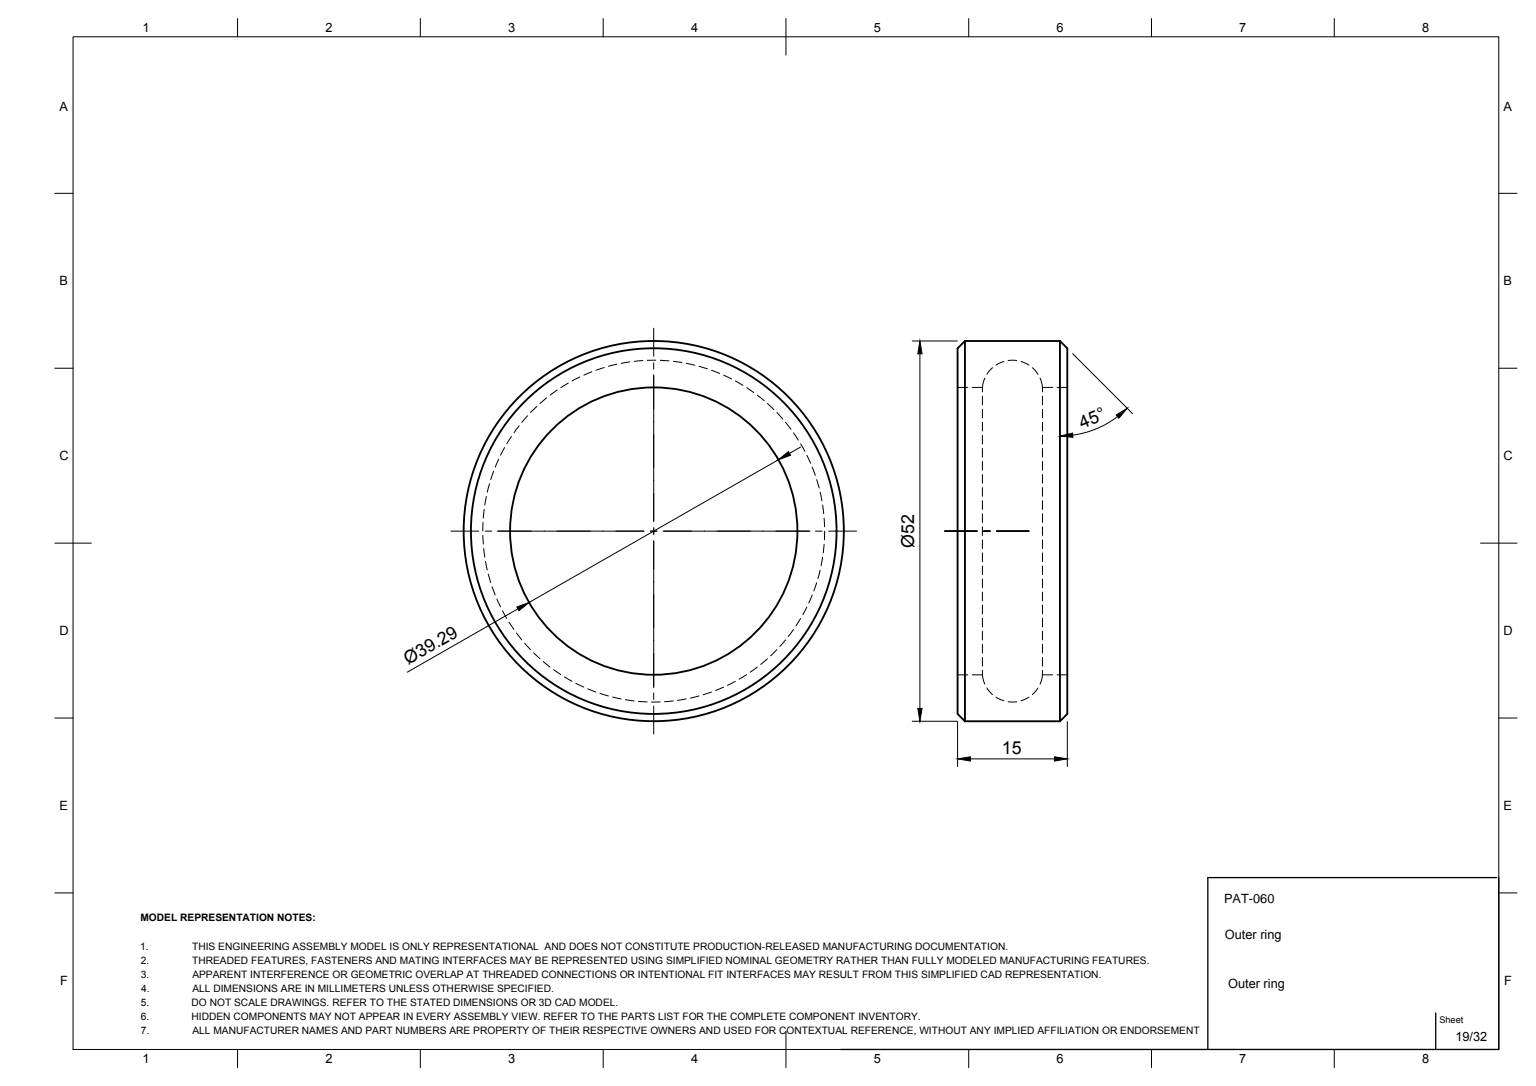
ISO-10303-21;
HEADER;
/* Generated by software containing ST-Developer
 * from STEP Tools, Inc. (www.steptools.com) 
 */

FILE_DESCRIPTION(
/* description */ ('Indexing fixture plate with plunger'),
/* implementation_level */ '2;1');

FILE_NAME(
/* name */ 'Outer ring.step',
/* time_stamp */ '2026-10-28T03:23:41-07:00',
/* author */ (''),
/* organization */ (''),
/* preprocessor_version */ 'ST-DEVELOPER v20.2',
/* originating_system */ 'Autodesk Translation Framework v15.17.0.0',
/* authorisation */ '');

FILE_SCHEMA (('AUTOMOTIVE_DESIGN { 1 0 10303 214 3 1 1 }'));
ENDSEC;

DATA;
#10=MECHANICAL_DESIGN_GEOMETRIC_PRESENTATION_REPRESENTATION('',(#331),#10020);
#214=TOROIDAL_SURFACE('',#5106,1.925,0.412776);
#220=CONICAL_SURFACE('',#5117,2.55,0.785398163397449);
#221=CONICAL_SURFACE('',#5121,2.55,0.785398163397449);
#277=SHAPE_REPRESENTATION_RELATIONSHIP('SRR','None',#10152,#304);
#304=ADVANCED_BREP_SHAPE_REPRESENTATION('',(#366),#10005);
#331=STYLED_ITEM('',(#10368),#366);
#366=MANIFOLD_SOLID_BREP('Body1',#4586);
#433=FACE_BOUND('',#1099,.T.);
#434=FACE_BOUND('',#1104,.T.);
#585=PLANE('',#5114);
#586=PLANE('',#5123);
#764=FACE_OUTER_BOUND('',#1096,.T.);
#765=FACE_OUTER_BOUND('',#1097,.T.);
#766=FACE_OUTER_BOUND('',#1098,.T.);
#767=FACE_OUTER_BOUND('',#1100,.T.);
#768=FACE_OUTER_BOUND('',#1101,.T.);
#769=FACE_OUTER_BOUND('',#1102,.T.);
#770=FACE_OUTER_BOUND('',#1103,.T.);
#771=FACE_OUTER_BOUND('',#1105,.T.);
#1096=EDGE_LOOP('',(#3403,#3404,#3405,#3406,#3407,#3408));
#1097=EDGE_LOOP('',(#3409,#3410,#3411,#3412,#3413));
#1098=EDGE_LOOP('',(#3414));
#1099=EDGE_LOOP('',(#3415));
#1100=EDGE_LOOP('',(#3416,#3417,#3418,#3419));
#1101=EDGE_LOOP('',(#3420,#3421,#3422,#3423));
#1102=EDGE_LOOP('',(#3424,#3425,#3426,#3427));
#1103=EDGE_LOOP('',(#3428));
#1104=EDGE_LOOP('',(#3429));
#1105=EDGE_LOOP('',(#3430,#3431,#3432,#3433,#3434));
#1468=LINE('',#8647,#1688);
#1469=LINE('',#8656,#1689);
#1470=LINE('',#8660,#1690);
#1471=LINE('',#8664,#1691);
#1472=LINE('',#8667,#1692);
#1688=VECTOR('',#6063,1.96469);
#1689=VECTOR('',#6074,2.55);
#1690=VECTOR('',#6079,2.6);
#1691=VECTOR('',#6084,2.55);
#1692=VECTOR('',#6089,1.96469);
#1920=CIRCLE('',#5107,1.96469);
#1921=CIRCLE('',#5108,1.96469);
#1922=CIRCLE('',#5109,0.412776);
#1923=CIRCLE('',#5110,1.96469);
#1924=CIRCLE('',#5111,1.96469);
#1925=CIRCLE('',#5113,1.96469);
#1926=CIRCLE('',#5115,2.5);
#1927=CIRCLE('',#5116,1.96469);
#1928=CIRCLE('',#5118,2.6);
#1929=CIRCLE('',#5120,2.6);
#1930=CIRCLE('',#5122,2.5);
#2247=VERTEX_POINT('',#8635);
#2248=VERTEX_POINT('',#8636);
#2249=VERTEX_POINT('',#8639);
#2250=VERTEX_POINT('',#8641);
#2251=VERTEX_POINT('',#8645);
#2252=VERTEX_POINT('',#8649);
#2253=VERTEX_POINT('',#8651);
#2254=VERTEX_POINT('',#8654);
#2255=VERTEX_POINT('',#8658);
#2256=VERTEX_POINT('',#8662);
#2681=EDGE_CURVE('',#2247,#2248,#1920,.T.);
#2682=EDGE_CURVE('',#2248,#2247,#1921,.T.);
#2683=EDGE_CURVE('',#2248,#2249,#1922,.T.);
#2684=EDGE_CURVE('',#2250,#2249,#1923,.T.);
#2685=EDGE_CURVE('',#2249,#2250,#1924,.T.);
#2686=EDGE_CURVE('',#2251,#2251,#1925,.T.);
#2687=EDGE_CURVE('',#2251,#2250,#1468,.T.);
#2688=EDGE_CURVE('',#2252,#2252,#1926,.T.);
#2689=EDGE_CURVE('',#2253,#2253,#1927,.T.);
#2690=EDGE_CURVE('',#2254,#2254,#1928,.T.);
#2691=EDGE_CURVE('',#2254,#2252,#1469,.T.);
#2692=EDGE_CURVE('',#2255,#2255,#1929,.T.);
#2693=EDGE_CURVE('',#2255,#2254,#1470,.T.);
#2694=EDGE_CURVE('',#2256,#2256,#1930,.T.);
#2695=EDGE_CURVE('',#2256,#2255,#1471,.T.);
#2696=EDGE_CURVE('',#2247,#2253,#1472,.T.);
#3403=ORIENTED_EDGE('',*,*,#2681,.F.);
#3404=ORIENTED_EDGE('',*,*,#2682,.F.);
#3405=ORIENTED_EDGE('',*,*,#2683,.T.);
#3406=ORIENTED_EDGE('',*,*,#2684,.F.);
#3407=ORIENTED_EDGE('',*,*,#2685,.F.);
#3408=ORIENTED_EDGE('',*,*,#2683,.F.);
#3409=ORIENTED_EDGE('',*,*,#2686,.T.);
#3410=ORIENTED_EDGE('',*,*,#2687,.T.);
#3411=ORIENTED_EDGE('',*,*,#2684,.T.);
#3412=ORIENTED_EDGE('',*,*,#2685,.T.);
#3413=ORIENTED_EDGE('',*,*,#2687,.F.);
#3414=ORIENTED_EDGE('',*,*,#2688,.F.);
#3415=ORIENTED_EDGE('',*,*,#2689,.T.);
#3416=ORIENTED_EDGE('',*,*,#2690,.F.);
#3417=ORIENTED_EDGE('',*,*,#2691,.T.);
#3418=ORIENTED_EDGE('',*,*,#2688,.T.);
#3419=ORIENTED_EDGE('',*,*,#2691,.F.);
#3420=ORIENTED_EDGE('',*,*,#2692,.F.);
#3421=ORIENTED_EDGE('',*,*,#2693,.T.);
#3422=ORIENTED_EDGE('',*,*,#2690,.T.);
#3423=ORIENTED_EDGE('',*,*,#2693,.F.);
#3424=ORIENTED_EDGE('',*,*,#2694,.F.);
#3425=ORIENTED_EDGE('',*,*,#2695,.T.);
#3426=ORIENTED_EDGE('',*,*,#2692,.T.);
#3427=ORIENTED_EDGE('',*,*,#2695,.F.);
#3428=ORIENTED_EDGE('',*,*,#2694,.T.);
#3429=ORIENTED_EDGE('',*,*,#2686,.F.);
#3430=ORIENTED_EDGE('',*,*,#2681,.T.);
#3431=ORIENTED_EDGE('',*,*,#2682,.T.);
#3432=ORIENTED_EDGE('',*,*,#2696,.T.);
#3433=ORIENTED_EDGE('',*,*,#2689,.F.);
#3434=ORIENTED_EDGE('',*,*,#2696,.F.);
#4206=CYLINDRICAL_SURFACE('',#5112,1.96469);
#4207=CYLINDRICAL_SURFACE('',#5119,2.6);
#4208=CYLINDRICAL_SURFACE('',#5124,1.96469);
#4379=ADVANCED_FACE('',(#764),#214,.F.);
#4380=ADVANCED_FACE('',(#765),#4206,.F.);
#4381=ADVANCED_FACE('',(#766,#433),#585,.T.);
#4382=ADVANCED_FACE('',(#767),#220,.T.);
#4383=ADVANCED_FACE('',(#768),#4207,.T.);
#4384=ADVANCED_FACE('',(#769),#221,.T.);
#4385=ADVANCED_FACE('',(#770,#434),#586,.T.);
#4386=ADVANCED_FACE('',(#771),#4208,.F.);
#4586=CLOSED_SHELL('',(#4379,#4380,#4381,#4382,#4383,#4384,#4385,#4386));
#5105=AXIS2_PLACEMENT_3D('',#8633,#6045,#6046);
#5106=AXIS2_PLACEMENT_3D('',#8634,#6047,#6048);
#5107=AXIS2_PLACEMENT_3D('',#8637,#6049,#6050);
#5108=AXIS2_PLACEMENT_3D('',#8638,#6051,#6052);
#5109=AXIS2_PLACEMENT_3D('',#8640,#6053,#6054);
#5110=AXIS2_PLACEMENT_3D('',#8642,#6055,#6056);
#5111=AXIS2_PLACEMENT_3D('',#8643,#6057,#6058);
#5112=AXIS2_PLACEMENT_3D('',#8644,#6059,#6060);
#5113=AXIS2_PLACEMENT_3D('',#8646,#6061,#6062);
#5114=AXIS2_PLACEMENT_3D('',#8648,#6064,#6065);
#5115=AXIS2_PLACEMENT_3D('',#8650,#6066,#6067);
#5116=AXIS2_PLACEMENT_3D('',#8652,#6068,#6069);
#5117=AXIS2_PLACEMENT_3D('',#8653,#6070,#6071);
#5118=AXIS2_PLACEMENT_3D('',#8655,#6072,#6073);
#5119=AXIS2_PLACEMENT_3D('',#8657,#6075,#6076);
#5120=AXIS2_PLACEMENT_3D('',#8659,#6077,#6078);
#5121=AXIS2_PLACEMENT_3D('',#8661,#6080,#6081);
#5122=AXIS2_PLACEMENT_3D('',#8663,#6082,#6083);
#5123=AXIS2_PLACEMENT_3D('',#8665,#6085,#6086);
#5124=AXIS2_PLACEMENT_3D('',#8666,#6087,#6088);
#6045=DIRECTION('axis',(0.,0.,1.));
#6046=DIRECTION('refdir',(1.,0.,0.));
#6047=DIRECTION('center_axis',(0.,-1.,0.));
#6048=DIRECTION('ref_axis',(0.,0.,-1.));
#6049=DIRECTION('center_axis',(0.,-1.,0.));
#6050=DIRECTION('ref_axis',(1.,0.,0.));
#6051=DIRECTION('center_axis',(0.,-1.,0.));
#6052=DIRECTION('ref_axis',(1.,0.,0.));
#6053=DIRECTION('center_axis',(1.,0.,1.22464679914735E-16));
#6054=DIRECTION('ref_axis',(-1.22464679914735E-16,0.,1.));
#6055=DIRECTION('center_axis',(0.,1.,0.));
#6056=DIRECTION('ref_axis',(1.,0.,0.));
#6057=DIRECTION('center_axis',(0.,1.,0.));
#6058=DIRECTION('ref_axis',(1.,0.,0.));
#6059=DIRECTION('center_axis',(0.,-1.,0.));
#6060=DIRECTION('ref_axis',(1.,0.,0.));
#6061=DIRECTION('center_axis',(0.,-1.,0.));
#6062=DIRECTION('ref_axis',(1.,0.,0.));
#6063=DIRECTION('',(0.,1.,0.));
#6064=DIRECTION('center_axis',(0.,1.,0.));
#6065=DIRECTION('ref_axis',(0.,0.,1.));
#6066=DIRECTION('center_axis',(0.,-1.,0.));
#6067=DIRECTION('ref_axis',(1.,0.,0.));
#6068=DIRECTION('center_axis',(0.,-1.,0.));
#6069=DIRECTION('ref_axis',(1.,0.,0.));
#6070=DIRECTION('center_axis',(0.,-1.,0.));
#6071=DIRECTION('ref_axis',(1.,0.,0.));
#6072=DIRECTION('center_axis',(0.,-1.,0.));
#6073=DIRECTION('ref_axis',(1.,0.,0.));
#6074=DIRECTION('',(0.707106781186548,0.707106781186547,8.65956056235494E-17));
#6075=DIRECTION('center_axis',(0.,-1.,0.));
#6076=DIRECTION('ref_axis',(1.,0.,0.));
#6077=DIRECTION('center_axis',(0.,-1.,0.));
#6078=DIRECTION('ref_axis',(1.,0.,0.));
#6079=DIRECTION('',(0.,1.,0.));
#6080=DIRECTION('center_axis',(0.,1.,0.));
#6081=DIRECTION('ref_axis',(1.,0.,0.));
#6082=DIRECTION('center_axis',(0.,-1.,0.));
#6083=DIRECTION('ref_axis',(1.,0.,0.));
#6084=DIRECTION('',(-0.707106781186548,0.707106781186547,-8.65956056235494E-17));
#6085=DIRECTION('center_axis',(0.,-1.,0.));
#6086=DIRECTION('ref_axis',(0.,0.,-1.));
#6087=DIRECTION('center_axis',(0.,-1.,0.));
#6088=DIRECTION('ref_axis',(1.,0.,0.));
#6089=DIRECTION('',(0.,1.,0.));
#8633=CARTESIAN_POINT('',(0.,0.,0.));
#8634=CARTESIAN_POINT('Origin',(0.,0.,0.));
#8635=CARTESIAN_POINT('',(-1.96469,0.410863395882378,-2.40605131981681E-16));
#8636=CARTESIAN_POINT('',(-2.40605131981681E-16,0.410863395882378,1.96469));
#8637=CARTESIAN_POINT('Origin',(0.,0.410863395882378,0.));
#8638=CARTESIAN_POINT('Origin',(0.,0.410863395882378,0.));
#8639=CARTESIAN_POINT('',(-2.40605131981681E-16,-0.410863395882378,1.96469));
#8640=CARTESIAN_POINT('Origin',(-2.35744508835865E-16,0.,1.925));
#8641=CARTESIAN_POINT('',(-1.96469,-0.410863395882378,2.40605131981681E-16));
#8642=CARTESIAN_POINT('Origin',(0.,-0.410863395882378,0.));
#8643=CARTESIAN_POINT('Origin',(0.,-0.410863395882378,0.));
#8644=CARTESIAN_POINT('Origin',(0.,0.,0.));
#8645=CARTESIAN_POINT('',(-1.96469,-0.75,-2.40605131981681E-16));
#8646=CARTESIAN_POINT('Origin',(0.,-0.75,0.));
#8647=CARTESIAN_POINT('',(-1.96469,0.,-2.40605131981681E-16));
#8648=CARTESIAN_POINT('Origin',(2.5,0.75,0.));
#8649=CARTESIAN_POINT('',(-2.5,0.75,-3.06161699786838E-16));
#8650=CARTESIAN_POINT('Origin',(0.,0.75,0.));
#8651=CARTESIAN_POINT('',(-1.96469,0.75,-2.40605131981681E-16));
#8652=CARTESIAN_POINT('Origin',(0.,0.75,0.));
#8653=CARTESIAN_POINT('Origin',(0.,0.7,0.));
#8654=CARTESIAN_POINT('',(-2.6,0.65,-3.18408167778312E-16));
#8655=CARTESIAN_POINT('Origin',(0.,0.65,0.));
#8656=CARTESIAN_POINT('',(-2.55,0.7,-3.12284933782575E-16));
#8657=CARTESIAN_POINT('Origin',(0.,0.,0.));
#8658=CARTESIAN_POINT('',(-2.6,-0.65,-3.18408167778312E-16));
#8659=CARTESIAN_POINT('Origin',(0.,-0.65,0.));
#8660=CARTESIAN_POINT('',(-2.6,0.,-3.18408167778312E-16));
#8661=CARTESIAN_POINT('Origin',(0.,-0.7,0.));
#8662=CARTESIAN_POINT('',(-2.5,-0.75,-3.06161699786838E-16));
#8663=CARTESIAN_POINT('Origin',(0.,-0.75,0.));
#8664=CARTESIAN_POINT('',(-2.55,-0.7,-3.12284933782575E-16));
#8665=CARTESIAN_POINT('Origin',(1.96469,-0.75,0.));
#8666=CARTESIAN_POINT('Origin',(0.,0.,0.));
#8667=CARTESIAN_POINT('',(-1.96469,0.,-2.40605131981681E-16));
#9972=UNCERTAINTY_MEASURE_WITH_UNIT(LENGTH_MEASURE(0.001),#10021,
'DISTANCE_ACCURACY_VALUE',
'Maximum model space distance between geometric entities at asserted c
onnectivities');
#9987=UNCERTAINTY_MEASURE_WITH_UNIT(LENGTH_MEASURE(0.001),#10021,
'DISTANCE_ACCURACY_VALUE',
'Maximum model space distance between geometric entities at asserted c
onnectivities');
#10005=(
GEOMETRIC_REPRESENTATION_CONTEXT(3)
GLOBAL_UNCERTAINTY_ASSIGNED_CONTEXT((#9972))
GLOBAL_UNIT_ASSIGNED_CONTEXT((#10021,#10023,#10024))
REPRESENTATION_CONTEXT('','3D')
);
#10020=(
GEOMETRIC_REPRESENTATION_CONTEXT(3)
GLOBAL_UNCERTAINTY_ASSIGNED_CONTEXT((#9987))
GLOBAL_UNIT_ASSIGNED_CONTEXT((#10021,#10023,#10024))
REPRESENTATION_CONTEXT('','3D')
);
#10021=(
LENGTH_UNIT()
NAMED_UNIT(*)
SI_UNIT(.CENTI.,.METRE.)
);
#10023=(
NAMED_UNIT(*)
PLANE_ANGLE_UNIT()
SI_UNIT($,.RADIAN.)
);
#10024=(
NAMED_UNIT(*)
SI_UNIT($,.STERADIAN.)
SOLID_ANGLE_UNIT()
);
#10042=SHAPE_DEFINITION_REPRESENTATION(#10074,#10152);
#10074=PRODUCT_DEFINITION_SHAPE('',$,#10185);
#10152=SHAPE_REPRESENTATION('',(#5105),#10005);
#10167=PRODUCT_DEFINITION_CONTEXT('part definition',#10265,'design');
#10185=PRODUCT_DEFINITION('Outer ring','Outer ring',#10217,#10167);
#10217=PRODUCT_DEFINITION_FORMATION('',$,#10284);
#10265=APPLICATION_CONTEXT(
'Core Data for Automotive Mechanical Design Process');
#10266=PRODUCT_CONTEXT('part definition',#10265,'mechanical');
#10284=PRODUCT('Outer ring','Outer ring','Outer ring',(#10266));
#10362=COLOUR_RGB('Grey',0.48,0.52,0.57);
#10363=FILL_AREA_STYLE_COLOUR('',#10362);
#10364=FILL_AREA_STYLE('',(#10363));
#10365=SURFACE_STYLE_FILL_AREA(#10364);
#10366=SURFACE_SIDE_STYLE('',(#10365));
#10367=SURFACE_STYLE_USAGE(.BOTH.,#10366);
#10368=PRESENTATION_STYLE_ASSIGNMENT((#10367));
ENDSEC;
END-ISO-10303-21;
